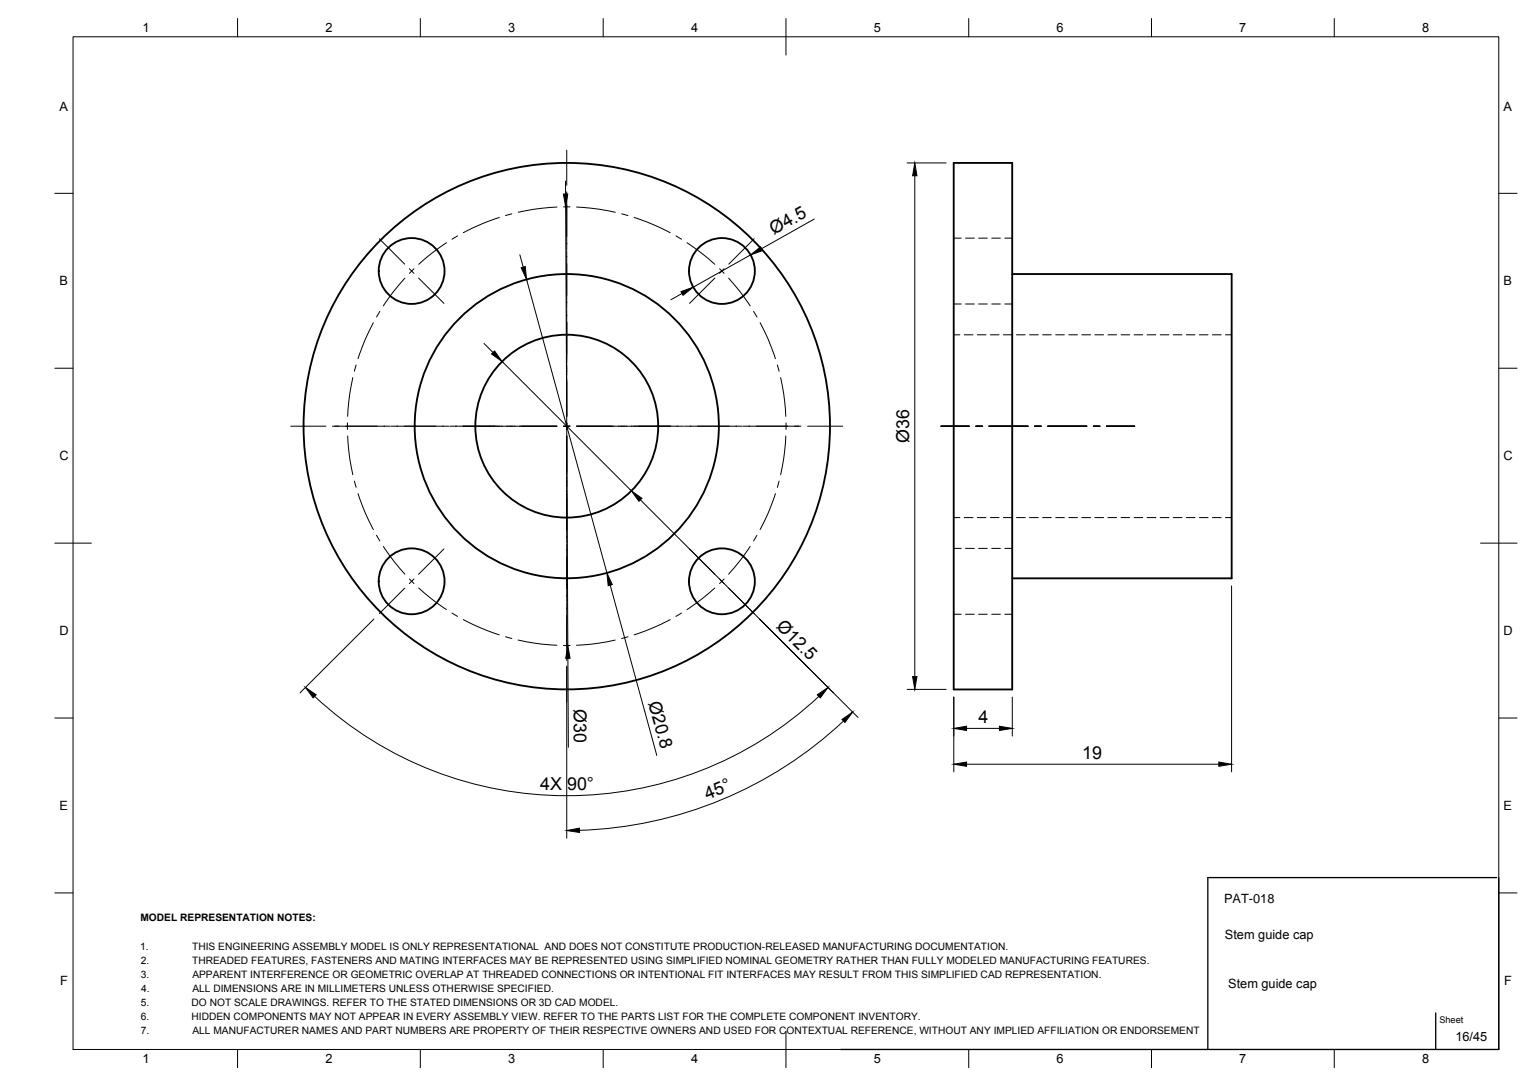
ISO-10303-21;
HEADER;
/* Generated by software containing ST-Developer
 * from STEP Tools, Inc. (www.steptools.com) 
 */

FILE_DESCRIPTION(
/* description */ ('Cam-driven reciprocating slide'),
/* implementation_level */ '2;1');

FILE_NAME(
/* name */ 'Stem guide cap.step',
/* time_stamp */ '2026-10-28T03:25:20-07:00',
/* author */ (''),
/* organization */ (''),
/* preprocessor_version */ 'ST-DEVELOPER v20.2',
/* originating_system */ 'Autodesk Translation Framework v15.17.0.0',
/* authorisation */ '');

FILE_SCHEMA (('AUTOMOTIVE_DESIGN { 1 0 10303 214 3 1 1 }'));
ENDSEC;

DATA;
#10=MECHANICAL_DESIGN_GEOMETRIC_PRESENTATION_REPRESENTATION('',(#433),#13277);
#359=SHAPE_REPRESENTATION_RELATIONSHIP('SRR','None',#13452,#396);
#396=ADVANCED_BREP_SHAPE_REPRESENTATION('',(#477),#13247);
#433=STYLED_ITEM('',(#13734),#477);
#477=MANIFOLD_SOLID_BREP('Body1',#6409);
#607=FACE_BOUND('',#1524,.T.);
#608=FACE_BOUND('',#1528,.T.);
#609=FACE_BOUND('',#1529,.T.);
#610=FACE_BOUND('',#1530,.T.);
#611=FACE_BOUND('',#1531,.T.);
#612=FACE_BOUND('',#1532,.T.);
#613=FACE_BOUND('',#1534,.T.);
#614=FACE_BOUND('',#1535,.T.);
#615=FACE_BOUND('',#1536,.T.);
#616=FACE_BOUND('',#1537,.T.);
#617=FACE_BOUND('',#1538,.T.);
#759=PLANE('',#7140);
#760=PLANE('',#7147);
#761=PLANE('',#7148);
#1039=FACE_OUTER_BOUND('',#1518,.T.);
#1040=FACE_OUTER_BOUND('',#1519,.T.);
#1041=FACE_OUTER_BOUND('',#1520,.T.);
#1042=FACE_OUTER_BOUND('',#1521,.T.);
#1043=FACE_OUTER_BOUND('',#1522,.T.);
#1044=FACE_OUTER_BOUND('',#1523,.T.);
#1045=FACE_OUTER_BOUND('',#1525,.T.);
#1046=FACE_OUTER_BOUND('',#1526,.T.);
#1047=FACE_OUTER_BOUND('',#1527,.T.);
#1048=FACE_OUTER_BOUND('',#1533,.T.);
#1518=EDGE_LOOP('',(#4960,#4961,#4962,#4963));
#1519=EDGE_LOOP('',(#4964,#4965,#4966,#4967));
#1520=EDGE_LOOP('',(#4968,#4969,#4970,#4971));
#1521=EDGE_LOOP('',(#4972,#4973,#4974,#4975));
#1522=EDGE_LOOP('',(#4976,#4977,#4978,#4979));
#1523=EDGE_LOOP('',(#4980));
#1524=EDGE_LOOP('',(#4981));
#1525=EDGE_LOOP('',(#4982,#4983,#4984,#4985));
#1526=EDGE_LOOP('',(#4986,#4987,#4988,#4989));
#1527=EDGE_LOOP('',(#4990));
#1528=EDGE_LOOP('',(#4991));
#1529=EDGE_LOOP('',(#4992));
#1530=EDGE_LOOP('',(#4993));
#1531=EDGE_LOOP('',(#4994));
#1532=EDGE_LOOP('',(#4995));
#1533=EDGE_LOOP('',(#4996));
#1534=EDGE_LOOP('',(#4997));
#1535=EDGE_LOOP('',(#4998));
#1536=EDGE_LOOP('',(#4999));
#1537=EDGE_LOOP('',(#5000));
#1538=EDGE_LOOP('',(#5001));
#2025=LINE('',#10416,#2464);
#2026=LINE('',#10422,#2465);
#2027=LINE('',#10428,#2466);
#2028=LINE('',#10434,#2467);
#2029=LINE('',#10440,#2468);
#2030=LINE('',#10448,#2469);
#2031=LINE('',#10453,#2470);
#2464=VECTOR('',#8409,0.225);
#2465=VECTOR('',#8416,0.225);
#2466=VECTOR('',#8423,0.225);
#2467=VECTOR('',#8430,0.225);
#2468=VECTOR('',#8437,1.04);
#2469=VECTOR('',#8448,0.625);
#2470=VECTOR('',#8453,1.8);
#2831=CIRCLE('',#7126,0.225);
#2832=CIRCLE('',#7127,0.225);
#2833=CIRCLE('',#7129,0.225);
#2834=CIRCLE('',#7130,0.225);
#2835=CIRCLE('',#7132,0.225);
#2836=CIRCLE('',#7133,0.225);
#2837=CIRCLE('',#7135,0.225);
#2838=CIRCLE('',#7136,0.225);
#2839=CIRCLE('',#7138,1.04);
#2840=CIRCLE('',#7139,1.04);
#2841=CIRCLE('',#7141,0.625);
#2842=CIRCLE('',#7143,0.625);
#2843=CIRCLE('',#7145,1.8);
#2844=CIRCLE('',#7146,1.8);
#3243=VERTEX_POINT('',#10413);
#3244=VERTEX_POINT('',#10415);
#3245=VERTEX_POINT('',#10419);
#3246=VERTEX_POINT('',#10421);
#3247=VERTEX_POINT('',#10425);
#3248=VERTEX_POINT('',#10427);
#3249=VERTEX_POINT('',#10431);
#3250=VERTEX_POINT('',#10433);
#3251=VERTEX_POINT('',#10437);
#3252=VERTEX_POINT('',#10439);
#3253=VERTEX_POINT('',#10443);
#3254=VERTEX_POINT('',#10446);
#3255=VERTEX_POINT('',#10450);
#3256=VERTEX_POINT('',#10452);
#3870=EDGE_CURVE('',#3243,#3243,#2831,.T.);
#3871=EDGE_CURVE('',#3243,#3244,#2025,.T.);
#3872=EDGE_CURVE('',#3244,#3244,#2832,.T.);
#3873=EDGE_CURVE('',#3245,#3245,#2833,.T.);
#3874=EDGE_CURVE('',#3245,#3246,#2026,.T.);
#3875=EDGE_CURVE('',#3246,#3246,#2834,.T.);
#3876=EDGE_CURVE('',#3247,#3247,#2835,.T.);
#3877=EDGE_CURVE('',#3247,#3248,#2027,.T.);
#3878=EDGE_CURVE('',#3248,#3248,#2836,.T.);
#3879=EDGE_CURVE('',#3249,#3249,#2837,.T.);
#3880=EDGE_CURVE('',#3249,#3250,#2028,.T.);
#3881=EDGE_CURVE('',#3250,#3250,#2838,.T.);
#3882=EDGE_CURVE('',#3251,#3251,#2839,.T.);
#3883=EDGE_CURVE('',#3251,#3252,#2029,.T.);
#3884=EDGE_CURVE('',#3252,#3252,#2840,.T.);
#3885=EDGE_CURVE('',#3253,#3253,#2841,.T.);
#3886=EDGE_CURVE('',#3254,#3254,#2842,.T.);
#3887=EDGE_CURVE('',#3254,#3253,#2030,.T.);
#3888=EDGE_CURVE('',#3255,#3255,#2843,.T.);
#3889=EDGE_CURVE('',#3255,#3256,#2031,.T.);
#3890=EDGE_CURVE('',#3256,#3256,#2844,.T.);
#4960=ORIENTED_EDGE('',*,*,#3870,.F.);
#4961=ORIENTED_EDGE('',*,*,#3871,.T.);
#4962=ORIENTED_EDGE('',*,*,#3872,.F.);
#4963=ORIENTED_EDGE('',*,*,#3871,.F.);
#4964=ORIENTED_EDGE('',*,*,#3873,.F.);
#4965=ORIENTED_EDGE('',*,*,#3874,.T.);
#4966=ORIENTED_EDGE('',*,*,#3875,.F.);
#4967=ORIENTED_EDGE('',*,*,#3874,.F.);
#4968=ORIENTED_EDGE('',*,*,#3876,.F.);
#4969=ORIENTED_EDGE('',*,*,#3877,.T.);
#4970=ORIENTED_EDGE('',*,*,#3878,.F.);
#4971=ORIENTED_EDGE('',*,*,#3877,.F.);
#4972=ORIENTED_EDGE('',*,*,#3879,.F.);
#4973=ORIENTED_EDGE('',*,*,#3880,.T.);
#4974=ORIENTED_EDGE('',*,*,#3881,.F.);
#4975=ORIENTED_EDGE('',*,*,#3880,.F.);
#4976=ORIENTED_EDGE('',*,*,#3882,.F.);
#4977=ORIENTED_EDGE('',*,*,#3883,.T.);
#4978=ORIENTED_EDGE('',*,*,#3884,.T.);
#4979=ORIENTED_EDGE('',*,*,#3883,.F.);
#4980=ORIENTED_EDGE('',*,*,#3884,.F.);
#4981=ORIENTED_EDGE('',*,*,#3885,.F.);
#4982=ORIENTED_EDGE('',*,*,#3886,.F.);
#4983=ORIENTED_EDGE('',*,*,#3887,.T.);
#4984=ORIENTED_EDGE('',*,*,#3885,.T.);
#4985=ORIENTED_EDGE('',*,*,#3887,.F.);
#4986=ORIENTED_EDGE('',*,*,#3888,.F.);
#4987=ORIENTED_EDGE('',*,*,#3889,.T.);
#4988=ORIENTED_EDGE('',*,*,#3890,.T.);
#4989=ORIENTED_EDGE('',*,*,#3889,.F.);
#4990=ORIENTED_EDGE('',*,*,#3888,.T.);
#4991=ORIENTED_EDGE('',*,*,#3886,.T.);
#4992=ORIENTED_EDGE('',*,*,#3881,.T.);
#4993=ORIENTED_EDGE('',*,*,#3878,.T.);
#4994=ORIENTED_EDGE('',*,*,#3875,.T.);
#4995=ORIENTED_EDGE('',*,*,#3872,.T.);
#4996=ORIENTED_EDGE('',*,*,#3890,.F.);
#4997=ORIENTED_EDGE('',*,*,#3882,.T.);
#4998=ORIENTED_EDGE('',*,*,#3879,.T.);
#4999=ORIENTED_EDGE('',*,*,#3876,.T.);
#5000=ORIENTED_EDGE('',*,*,#3873,.T.);
#5001=ORIENTED_EDGE('',*,*,#3870,.T.);
#5952=CYLINDRICAL_SURFACE('',#7125,0.225);
#5953=CYLINDRICAL_SURFACE('',#7128,0.225);
#5954=CYLINDRICAL_SURFACE('',#7131,0.225);
#5955=CYLINDRICAL_SURFACE('',#7134,0.225);
#5956=CYLINDRICAL_SURFACE('',#7137,1.04);
#5957=CYLINDRICAL_SURFACE('',#7142,0.625);
#5958=CYLINDRICAL_SURFACE('',#7144,1.8);
#6157=ADVANCED_FACE('',(#1039),#5952,.F.);
#6158=ADVANCED_FACE('',(#1040),#5953,.F.);
#6159=ADVANCED_FACE('',(#1041),#5954,.F.);
#6160=ADVANCED_FACE('',(#1042),#5955,.F.);
#6161=ADVANCED_FACE('',(#1043),#5956,.T.);
#6162=ADVANCED_FACE('',(#1044,#607),#759,.F.);
#6163=ADVANCED_FACE('',(#1045),#5957,.F.);
#6164=ADVANCED_FACE('',(#1046),#5958,.T.);
#6165=ADVANCED_FACE('',(#1047,#608,#609,#610,#611,#612),#760,.T.);
#6166=ADVANCED_FACE('',(#1048,#613,#614,#615,#616,#617),#761,.F.);
#6409=CLOSED_SHELL('',(#6157,#6158,#6159,#6160,#6161,#6162,#6163,#6164,
#6165,#6166));
#7124=AXIS2_PLACEMENT_3D('',#10411,#8403,#8404);
#7125=AXIS2_PLACEMENT_3D('',#10412,#8405,#8406);
#7126=AXIS2_PLACEMENT_3D('',#10414,#8407,#8408);
#7127=AXIS2_PLACEMENT_3D('',#10417,#8410,#8411);
#7128=AXIS2_PLACEMENT_3D('',#10418,#8412,#8413);
#7129=AXIS2_PLACEMENT_3D('',#10420,#8414,#8415);
#7130=AXIS2_PLACEMENT_3D('',#10423,#8417,#8418);
#7131=AXIS2_PLACEMENT_3D('',#10424,#8419,#8420);
#7132=AXIS2_PLACEMENT_3D('',#10426,#8421,#8422);
#7133=AXIS2_PLACEMENT_3D('',#10429,#8424,#8425);
#7134=AXIS2_PLACEMENT_3D('',#10430,#8426,#8427);
#7135=AXIS2_PLACEMENT_3D('',#10432,#8428,#8429);
#7136=AXIS2_PLACEMENT_3D('',#10435,#8431,#8432);
#7137=AXIS2_PLACEMENT_3D('',#10436,#8433,#8434);
#7138=AXIS2_PLACEMENT_3D('',#10438,#8435,#8436);
#7139=AXIS2_PLACEMENT_3D('',#10441,#8438,#8439);
#7140=AXIS2_PLACEMENT_3D('',#10442,#8440,#8441);
#7141=AXIS2_PLACEMENT_3D('',#10444,#8442,#8443);
#7142=AXIS2_PLACEMENT_3D('',#10445,#8444,#8445);
#7143=AXIS2_PLACEMENT_3D('',#10447,#8446,#8447);
#7144=AXIS2_PLACEMENT_3D('',#10449,#8449,#8450);
#7145=AXIS2_PLACEMENT_3D('',#10451,#8451,#8452);
#7146=AXIS2_PLACEMENT_3D('',#10454,#8454,#8455);
#7147=AXIS2_PLACEMENT_3D('',#10455,#8456,#8457);
#7148=AXIS2_PLACEMENT_3D('',#10456,#8458,#8459);
#8403=DIRECTION('axis',(0.,0.,1.));
#8404=DIRECTION('refdir',(1.,0.,0.));
#8405=DIRECTION('center_axis',(0.,0.,1.));
#8406=DIRECTION('ref_axis',(1.,0.,0.));
#8407=DIRECTION('center_axis',(0.,0.,1.));
#8408=DIRECTION('ref_axis',(1.,0.,0.));
#8409=DIRECTION('',(0.,0.,1.));
#8410=DIRECTION('center_axis',(0.,0.,-1.));
#8411=DIRECTION('ref_axis',(1.,0.,0.));
#8412=DIRECTION('center_axis',(0.,0.,1.));
#8413=DIRECTION('ref_axis',(1.,0.,0.));
#8414=DIRECTION('center_axis',(0.,0.,1.));
#8415=DIRECTION('ref_axis',(1.,0.,0.));
#8416=DIRECTION('',(0.,0.,1.));
#8417=DIRECTION('center_axis',(0.,0.,-1.));
#8418=DIRECTION('ref_axis',(1.,0.,0.));
#8419=DIRECTION('center_axis',(0.,0.,1.));
#8420=DIRECTION('ref_axis',(1.,0.,0.));
#8421=DIRECTION('center_axis',(0.,0.,1.));
#8422=DIRECTION('ref_axis',(1.,0.,0.));
#8423=DIRECTION('',(0.,0.,1.));
#8424=DIRECTION('center_axis',(0.,0.,-1.));
#8425=DIRECTION('ref_axis',(1.,0.,0.));
#8426=DIRECTION('center_axis',(0.,0.,1.));
#8427=DIRECTION('ref_axis',(1.,0.,0.));
#8428=DIRECTION('center_axis',(0.,0.,1.));
#8429=DIRECTION('ref_axis',(1.,0.,0.));
#8430=DIRECTION('',(0.,0.,1.));
#8431=DIRECTION('center_axis',(0.,0.,-1.));
#8432=DIRECTION('ref_axis',(1.,0.,0.));
#8433=DIRECTION('center_axis',(0.,0.,1.));
#8434=DIRECTION('ref_axis',(1.,0.,0.));
#8435=DIRECTION('center_axis',(0.,0.,1.));
#8436=DIRECTION('ref_axis',(1.,0.,0.));
#8437=DIRECTION('',(0.,0.,-1.));
#8438=DIRECTION('center_axis',(0.,0.,1.));
#8439=DIRECTION('ref_axis',(1.,0.,0.));
#8440=DIRECTION('center_axis',(0.,0.,1.));
#8441=DIRECTION('ref_axis',(1.,0.,0.));
#8442=DIRECTION('center_axis',(0.,0.,-1.));
#8443=DIRECTION('ref_axis',(1.,0.,0.));
#8444=DIRECTION('center_axis',(0.,0.,1.));
#8445=DIRECTION('ref_axis',(1.,0.,0.));
#8446=DIRECTION('center_axis',(0.,0.,-1.));
#8447=DIRECTION('ref_axis',(1.,0.,0.));
#8448=DIRECTION('',(0.,0.,-1.));
#8449=DIRECTION('center_axis',(0.,0.,1.));
#8450=DIRECTION('ref_axis',(1.,0.,0.));
#8451=DIRECTION('center_axis',(0.,0.,1.));
#8452=DIRECTION('ref_axis',(1.,0.,0.));
#8453=DIRECTION('',(0.,0.,-1.));
#8454=DIRECTION('center_axis',(0.,0.,1.));
#8455=DIRECTION('ref_axis',(1.,0.,0.));
#8456=DIRECTION('center_axis',(0.,0.,1.));
#8457=DIRECTION('ref_axis',(1.,0.,0.));
#8458=DIRECTION('center_axis',(0.,0.,1.));
#8459=DIRECTION('ref_axis',(1.,0.,0.));
#10411=CARTESIAN_POINT('',(0.,0.,0.));
#10412=CARTESIAN_POINT('Origin',(-1.06066017177982,-1.06066017177982,20.9));
#10413=CARTESIAN_POINT('',(-1.28566017177982,-1.06066017177982,21.));
#10414=CARTESIAN_POINT('Origin',(-1.06066017177982,-1.06066017177982,21.));
#10415=CARTESIAN_POINT('',(-1.28566017177982,-1.06066017177982,21.4));
#10416=CARTESIAN_POINT('',(-1.28566017177982,-1.06066017177982,20.9));
#10417=CARTESIAN_POINT('Origin',(-1.06066017177982,-1.06066017177982,21.4));
#10418=CARTESIAN_POINT('Origin',(-1.06066017177982,1.06066017177982,20.9));
#10419=CARTESIAN_POINT('',(-1.28566017177982,1.06066017177982,21.));
#10420=CARTESIAN_POINT('Origin',(-1.06066017177982,1.06066017177982,21.));
#10421=CARTESIAN_POINT('',(-1.28566017177982,1.06066017177982,21.4));
#10422=CARTESIAN_POINT('',(-1.28566017177982,1.06066017177982,20.9));
#10423=CARTESIAN_POINT('Origin',(-1.06066017177982,1.06066017177982,21.4));
#10424=CARTESIAN_POINT('Origin',(1.06066017177982,1.06066017177982,20.9));
#10425=CARTESIAN_POINT('',(0.835660171779821,1.06066017177982,21.));
#10426=CARTESIAN_POINT('Origin',(1.06066017177982,1.06066017177982,21.));
#10427=CARTESIAN_POINT('',(0.835660171779821,1.06066017177982,21.4));
#10428=CARTESIAN_POINT('',(0.835660171779821,1.06066017177982,20.9));
#10429=CARTESIAN_POINT('Origin',(1.06066017177982,1.06066017177982,21.4));
#10430=CARTESIAN_POINT('Origin',(1.06066017177982,-1.06066017177982,20.9));
#10431=CARTESIAN_POINT('',(0.835660171779821,-1.06066017177982,21.));
#10432=CARTESIAN_POINT('Origin',(1.06066017177982,-1.06066017177982,21.));
#10433=CARTESIAN_POINT('',(0.835660171779821,-1.06066017177982,21.4));
#10434=CARTESIAN_POINT('',(0.835660171779821,-1.06066017177982,20.9));
#10435=CARTESIAN_POINT('Origin',(1.06066017177982,-1.06066017177982,21.4));
#10436=CARTESIAN_POINT('Origin',(0.,0.,19.5));
#10437=CARTESIAN_POINT('',(-1.04,-1.27363267111325E-16,21.));
#10438=CARTESIAN_POINT('Origin',(0.,0.,21.));
#10439=CARTESIAN_POINT('',(-1.04,-1.27363267111325E-16,19.5));
#10440=CARTESIAN_POINT('',(-1.04,-1.27363267111325E-16,19.5));
#10441=CARTESIAN_POINT('Origin',(0.,0.,19.5));
#10442=CARTESIAN_POINT('Origin',(0.,0.,19.5));
#10443=CARTESIAN_POINT('',(-0.625,-7.65404249467096E-17,19.5));
#10444=CARTESIAN_POINT('Origin',(0.,0.,19.5));
#10445=CARTESIAN_POINT('Origin',(0.,0.,21.));
#10446=CARTESIAN_POINT('',(-0.625,-7.65404249467096E-17,21.4));
#10447=CARTESIAN_POINT('Origin',(0.,0.,21.4));
#10448=CARTESIAN_POINT('',(-0.625,-7.65404249467096E-17,21.));
#10449=CARTESIAN_POINT('Origin',(0.,0.,21.));
#10450=CARTESIAN_POINT('',(-1.8,-2.20436423846524E-16,21.4));
#10451=CARTESIAN_POINT('Origin',(0.,0.,21.4));
#10452=CARTESIAN_POINT('',(-1.8,-2.20436423846524E-16,21.));
#10453=CARTESIAN_POINT('',(-1.8,-2.20436423846524E-16,21.));
#10454=CARTESIAN_POINT('Origin',(0.,0.,21.));
#10455=CARTESIAN_POINT('Origin',(0.,0.,21.4));
#10456=CARTESIAN_POINT('Origin',(0.,0.,21.));
#13203=UNCERTAINTY_MEASURE_WITH_UNIT(LENGTH_MEASURE(0.001),#13278,
'DISTANCE_ACCURACY_VALUE',
'Maximum model space distance between geometric entities at asserted c
onnectivities');
#13233=UNCERTAINTY_MEASURE_WITH_UNIT(LENGTH_MEASURE(0.001),#13278,
'DISTANCE_ACCURACY_VALUE',
'Maximum model space distance between geometric entities at asserted c
onnectivities');
#13247=(
GEOMETRIC_REPRESENTATION_CONTEXT(3)
GLOBAL_UNCERTAINTY_ASSIGNED_CONTEXT((#13203))
GLOBAL_UNIT_ASSIGNED_CONTEXT((#13278,#13280,#13281))
REPRESENTATION_CONTEXT('','3D')
);
#13277=(
GEOMETRIC_REPRESENTATION_CONTEXT(3)
GLOBAL_UNCERTAINTY_ASSIGNED_CONTEXT((#13233))
GLOBAL_UNIT_ASSIGNED_CONTEXT((#13278,#13280,#13281))
REPRESENTATION_CONTEXT('','3D')
);
#13278=(
LENGTH_UNIT()
NAMED_UNIT(*)
SI_UNIT(.CENTI.,.METRE.)
);
#13280=(
NAMED_UNIT(*)
PLANE_ANGLE_UNIT()
SI_UNIT($,.RADIAN.)
);
#13281=(
NAMED_UNIT(*)
SI_UNIT($,.STERADIAN.)
SOLID_ANGLE_UNIT()
);
#13295=SHAPE_DEFINITION_REPRESENTATION(#13338,#13452);
#13338=PRODUCT_DEFINITION_SHAPE('',$,#13496);
#13452=SHAPE_REPRESENTATION('',(#7124),#13247);
#13482=PRODUCT_DEFINITION_CONTEXT('part definition',#13613,'design');
#13496=PRODUCT_DEFINITION('Stem guide cap','Stem guide cap',#13539,#13482);
#13539=PRODUCT_DEFINITION_FORMATION('',$,#13628);
#13613=APPLICATION_CONTEXT(
'Core Data for Automotive Mechanical Design Process');
#13614=PRODUCT_CONTEXT('part definition',#13613,'mechanical');
#13628=PRODUCT('Stem guide cap','Stem guide cap','Stem guide cap',(#13614));
#13728=COLOUR_RGB('Off White',0.89,0.88,0.83);
#13729=FILL_AREA_STYLE_COLOUR('',#13728);
#13730=FILL_AREA_STYLE('',(#13729));
#13731=SURFACE_STYLE_FILL_AREA(#13730);
#13732=SURFACE_SIDE_STYLE('',(#13731));
#13733=SURFACE_STYLE_USAGE(.BOTH.,#13732);
#13734=PRESENTATION_STYLE_ASSIGNMENT((#13733));
ENDSEC;
END-ISO-10303-21;
